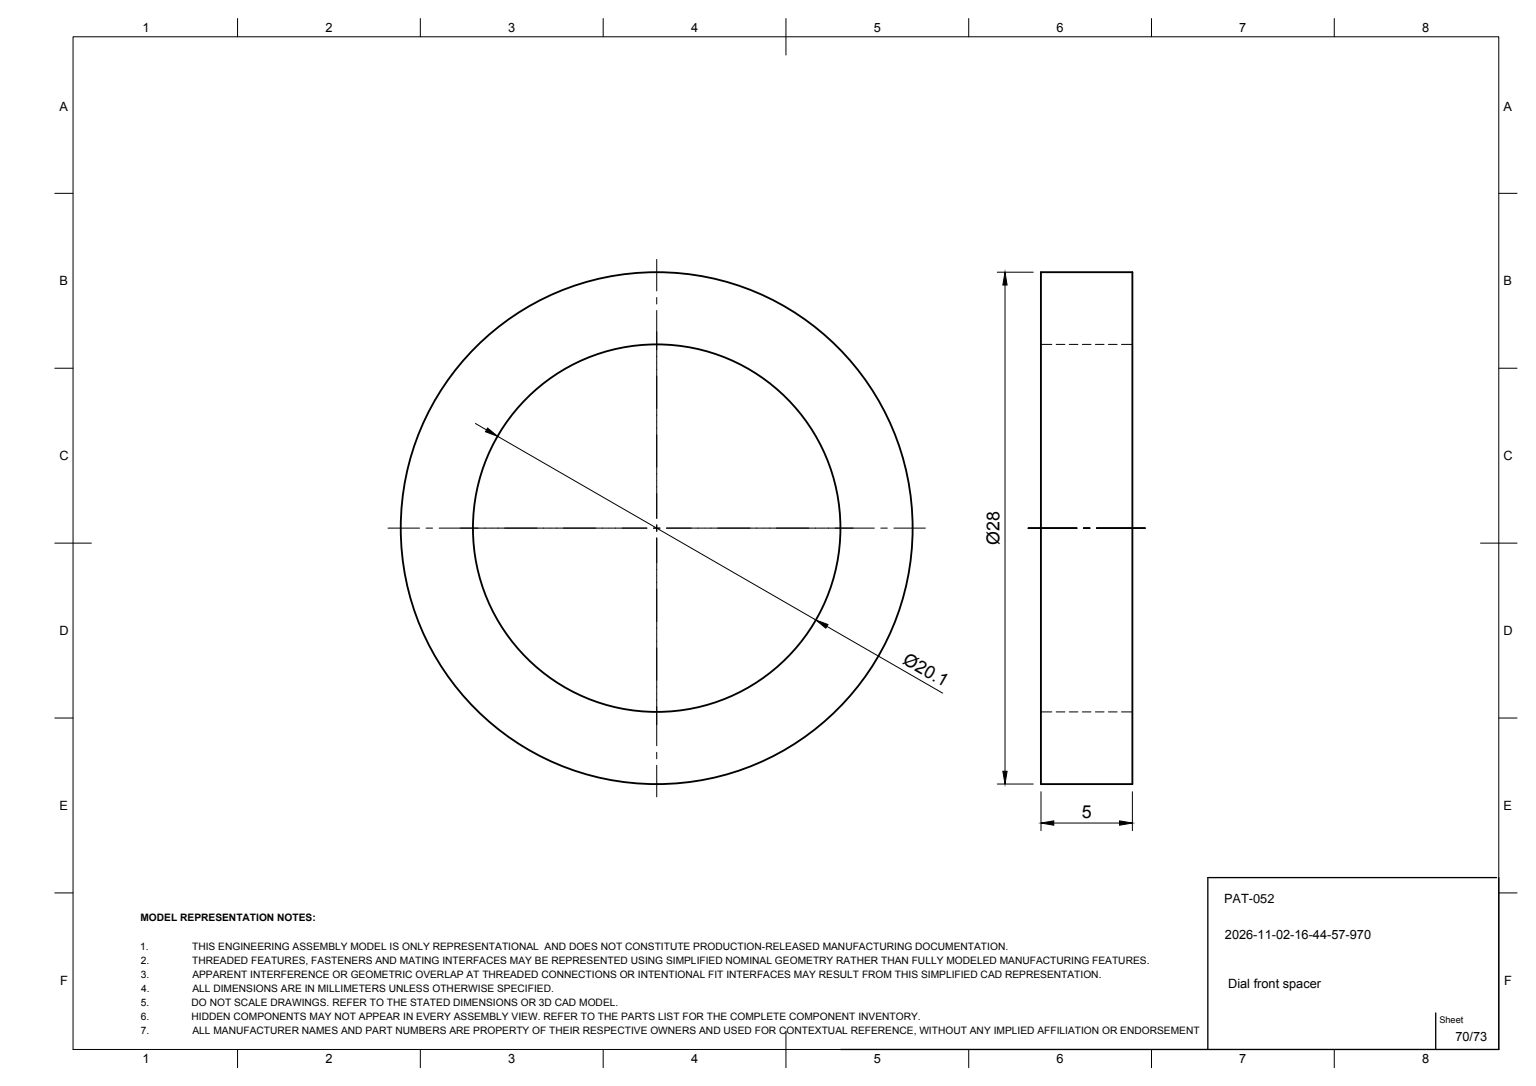
ISO-10303-21;
HEADER;
/* Generated by software containing ST-Developer
 * from STEP Tools, Inc. (www.steptools.com) 
 */

FILE_DESCRIPTION(
/* description */ ('Hand-crank gear train demonstrator'),
/* implementation_level */ '2;1');

FILE_NAME(
/* name */ 'Dial front spacer.step',
/* time_stamp */ '2026-10-28T03:22:13-07:00',
/* author */ (''),
/* organization */ (''),
/* preprocessor_version */ 'ST-DEVELOPER v20.2',
/* originating_system */ 'Autodesk Translation Framework v15.17.0.0',
/* authorisation */ '');

FILE_SCHEMA (('AUTOMOTIVE_DESIGN { 1 0 10303 214 3 1 1 }'));
ENDSEC;

DATA;
#10=MECHANICAL_DESIGN_GEOMETRIC_PRESENTATION_REPRESENTATION('',(#1260),#62758);
#1117=SHAPE_REPRESENTATION_RELATIONSHIP('SRR','None',#63095,#1181);
#1181=ADVANCED_BREP_SHAPE_REPRESENTATION('',(#1335),#62749);
#1260=STYLED_ITEM('',(#63455),#1335);
#1335=MANIFOLD_SOLID_BREP('Body1',#16444);
#1617=FACE_BOUND('',#4043,.T.);
#1618=FACE_BOUND('',#4045,.T.);
#2033=PLANE('',#18450);
#2034=PLANE('',#18451);
#2829=FACE_OUTER_BOUND('',#4040,.T.);
#2830=FACE_OUTER_BOUND('',#4041,.T.);
#2831=FACE_OUTER_BOUND('',#4042,.T.);
#2832=FACE_OUTER_BOUND('',#4044,.T.);
#4040=EDGE_LOOP('',(#13929,#13930,#13931,#13932));
#4041=EDGE_LOOP('',(#13933,#13934,#13935,#13936));
#4042=EDGE_LOOP('',(#13937));
#4043=EDGE_LOOP('',(#13938));
#4044=EDGE_LOOP('',(#13939));
#4045=EDGE_LOOP('',(#13940));
#5160=LINE('',#38623,#6292);
#5161=LINE('',#38629,#6293);
#6292=VECTOR('',#22281,1.005);
#6293=VECTOR('',#22288,1.4);
#7095=CIRCLE('',#18445,1.005);
#7096=CIRCLE('',#18446,1.005);
#7097=CIRCLE('',#18448,1.4);
#7098=CIRCLE('',#18449,1.4);
#8258=VERTEX_POINT('',#38620);
#8259=VERTEX_POINT('',#38622);
#8260=VERTEX_POINT('',#38626);
#8261=VERTEX_POINT('',#38628);
#10216=EDGE_CURVE('',#8258,#8258,#7095,.T.);
#10217=EDGE_CURVE('',#8258,#8259,#5160,.T.);
#10218=EDGE_CURVE('',#8259,#8259,#7096,.T.);
#10219=EDGE_CURVE('',#8260,#8260,#7097,.T.);
#10220=EDGE_CURVE('',#8260,#8261,#5161,.T.);
#10221=EDGE_CURVE('',#8261,#8261,#7098,.T.);
#13929=ORIENTED_EDGE('',*,*,#10216,.F.);
#13930=ORIENTED_EDGE('',*,*,#10217,.T.);
#13931=ORIENTED_EDGE('',*,*,#10218,.T.);
#13932=ORIENTED_EDGE('',*,*,#10217,.F.);
#13933=ORIENTED_EDGE('',*,*,#10219,.F.);
#13934=ORIENTED_EDGE('',*,*,#10220,.T.);
#13935=ORIENTED_EDGE('',*,*,#10221,.T.);
#13936=ORIENTED_EDGE('',*,*,#10220,.F.);
#13937=ORIENTED_EDGE('',*,*,#10219,.T.);
#13938=ORIENTED_EDGE('',*,*,#10216,.T.);
#13939=ORIENTED_EDGE('',*,*,#10221,.F.);
#13940=ORIENTED_EDGE('',*,*,#10218,.F.);
#15379=CYLINDRICAL_SURFACE('',#18444,1.005);
#15380=CYLINDRICAL_SURFACE('',#18447,1.4);
#16139=ADVANCED_FACE('',(#2829),#15379,.F.);
#16140=ADVANCED_FACE('',(#2830),#15380,.T.);
#16141=ADVANCED_FACE('',(#2831,#1617),#2033,.T.);
#16142=ADVANCED_FACE('',(#2832,#1618),#2034,.F.);
#16444=CLOSED_SHELL('',(#16139,#16140,#16141,#16142));
#18443=AXIS2_PLACEMENT_3D('',#38618,#22275,#22276);
#18444=AXIS2_PLACEMENT_3D('',#38619,#22277,#22278);
#18445=AXIS2_PLACEMENT_3D('',#38621,#22279,#22280);
#18446=AXIS2_PLACEMENT_3D('',#38624,#22282,#22283);
#18447=AXIS2_PLACEMENT_3D('',#38625,#22284,#22285);
#18448=AXIS2_PLACEMENT_3D('',#38627,#22286,#22287);
#18449=AXIS2_PLACEMENT_3D('',#38630,#22289,#22290);
#18450=AXIS2_PLACEMENT_3D('',#38631,#22291,#22292);
#18451=AXIS2_PLACEMENT_3D('',#38632,#22293,#22294);
#22275=DIRECTION('axis',(0.,0.,1.));
#22276=DIRECTION('refdir',(1.,0.,0.));
#22277=DIRECTION('center_axis',(0.,1.,0.));
#22278=DIRECTION('ref_axis',(1.,0.,0.));
#22279=DIRECTION('center_axis',(0.,-1.,0.));
#22280=DIRECTION('ref_axis',(1.,0.,0.));
#22281=DIRECTION('',(0.,-1.,0.));
#22282=DIRECTION('center_axis',(0.,-1.,0.));
#22283=DIRECTION('ref_axis',(1.,0.,0.));
#22284=DIRECTION('center_axis',(0.,1.,0.));
#22285=DIRECTION('ref_axis',(1.,0.,0.));
#22286=DIRECTION('center_axis',(0.,1.,0.));
#22287=DIRECTION('ref_axis',(1.,0.,0.));
#22288=DIRECTION('',(0.,-1.,0.));
#22289=DIRECTION('center_axis',(0.,1.,0.));
#22290=DIRECTION('ref_axis',(1.,0.,0.));
#22291=DIRECTION('center_axis',(0.,1.,0.));
#22292=DIRECTION('ref_axis',(1.,0.,0.));
#22293=DIRECTION('center_axis',(0.,1.,0.));
#22294=DIRECTION('ref_axis',(1.,0.,0.));
#38618=CARTESIAN_POINT('',(0.,0.,0.));
#38619=CARTESIAN_POINT('Origin',(18.,5.5,9.));
#38620=CARTESIAN_POINT('',(16.995,6.,9.));
#38621=CARTESIAN_POINT('Origin',(18.,6.,9.));
#38622=CARTESIAN_POINT('',(16.995,5.5,9.));
#38623=CARTESIAN_POINT('',(16.995,5.5,9.));
#38624=CARTESIAN_POINT('Origin',(18.,5.5,9.));
#38625=CARTESIAN_POINT('Origin',(18.,5.5,9.));
#38626=CARTESIAN_POINT('',(16.6,6.,9.));
#38627=CARTESIAN_POINT('Origin',(18.,6.,9.));
#38628=CARTESIAN_POINT('',(16.6,5.5,9.));
#38629=CARTESIAN_POINT('',(16.6,5.5,9.));
#38630=CARTESIAN_POINT('Origin',(18.,5.5,9.));
#38631=CARTESIAN_POINT('Origin',(18.,6.,9.));
#38632=CARTESIAN_POINT('Origin',(18.,5.5,9.));
#62675=UNCERTAINTY_MEASURE_WITH_UNIT(LENGTH_MEASURE(0.001),#62759,
'DISTANCE_ACCURACY_VALUE',
'Maximum model space distance between geometric entities at asserted c
onnectivities');
#62684=UNCERTAINTY_MEASURE_WITH_UNIT(LENGTH_MEASURE(0.001),#62759,
'DISTANCE_ACCURACY_VALUE',
'Maximum model space distance between geometric entities at asserted c
onnectivities');
#62749=(
GEOMETRIC_REPRESENTATION_CONTEXT(3)
GLOBAL_UNCERTAINTY_ASSIGNED_CONTEXT((#62675))
GLOBAL_UNIT_ASSIGNED_CONTEXT((#62759,#62761,#62762))
REPRESENTATION_CONTEXT('','3D')
);
#62758=(
GEOMETRIC_REPRESENTATION_CONTEXT(3)
GLOBAL_UNCERTAINTY_ASSIGNED_CONTEXT((#62684))
GLOBAL_UNIT_ASSIGNED_CONTEXT((#62759,#62761,#62762))
REPRESENTATION_CONTEXT('','3D')
);
#62759=(
LENGTH_UNIT()
NAMED_UNIT(*)
SI_UNIT(.CENTI.,.METRE.)
);
#62761=(
NAMED_UNIT(*)
PLANE_ANGLE_UNIT()
SI_UNIT($,.RADIAN.)
);
#62762=(
NAMED_UNIT(*)
SI_UNIT($,.STERADIAN.)
SOLID_ANGLE_UNIT()
);
#62827=SHAPE_DEFINITION_REPRESENTATION(#62910,#63095);
#62910=PRODUCT_DEFINITION_SHAPE('',$,#63169);
#63095=SHAPE_REPRESENTATION('',(#18443),#62749);
#63104=PRODUCT_DEFINITION_CONTEXT('part definition',#63325,'design');
#63169=PRODUCT_DEFINITION('Dial front spacer','Dial front spacer',#63242,
#63104);
#63242=PRODUCT_DEFINITION_FORMATION('',$,#63391);
#63325=APPLICATION_CONTEXT(
'Core Data for Automotive Mechanical Design Process');
#63326=PRODUCT_CONTEXT('part definition',#63325,'mechanical');
#63391=PRODUCT('Dial front spacer','Dial front spacer',
'Dial front spacer',(#63326));
#63449=COLOUR_RGB('Sky Blue',0.24,0.69,0.87);
#63450=FILL_AREA_STYLE_COLOUR('',#63449);
#63451=FILL_AREA_STYLE('',(#63450));
#63452=SURFACE_STYLE_FILL_AREA(#63451);
#63453=SURFACE_SIDE_STYLE('',(#63452));
#63454=SURFACE_STYLE_USAGE(.BOTH.,#63453);
#63455=PRESENTATION_STYLE_ASSIGNMENT((#63454));
ENDSEC;
END-ISO-10303-21;
